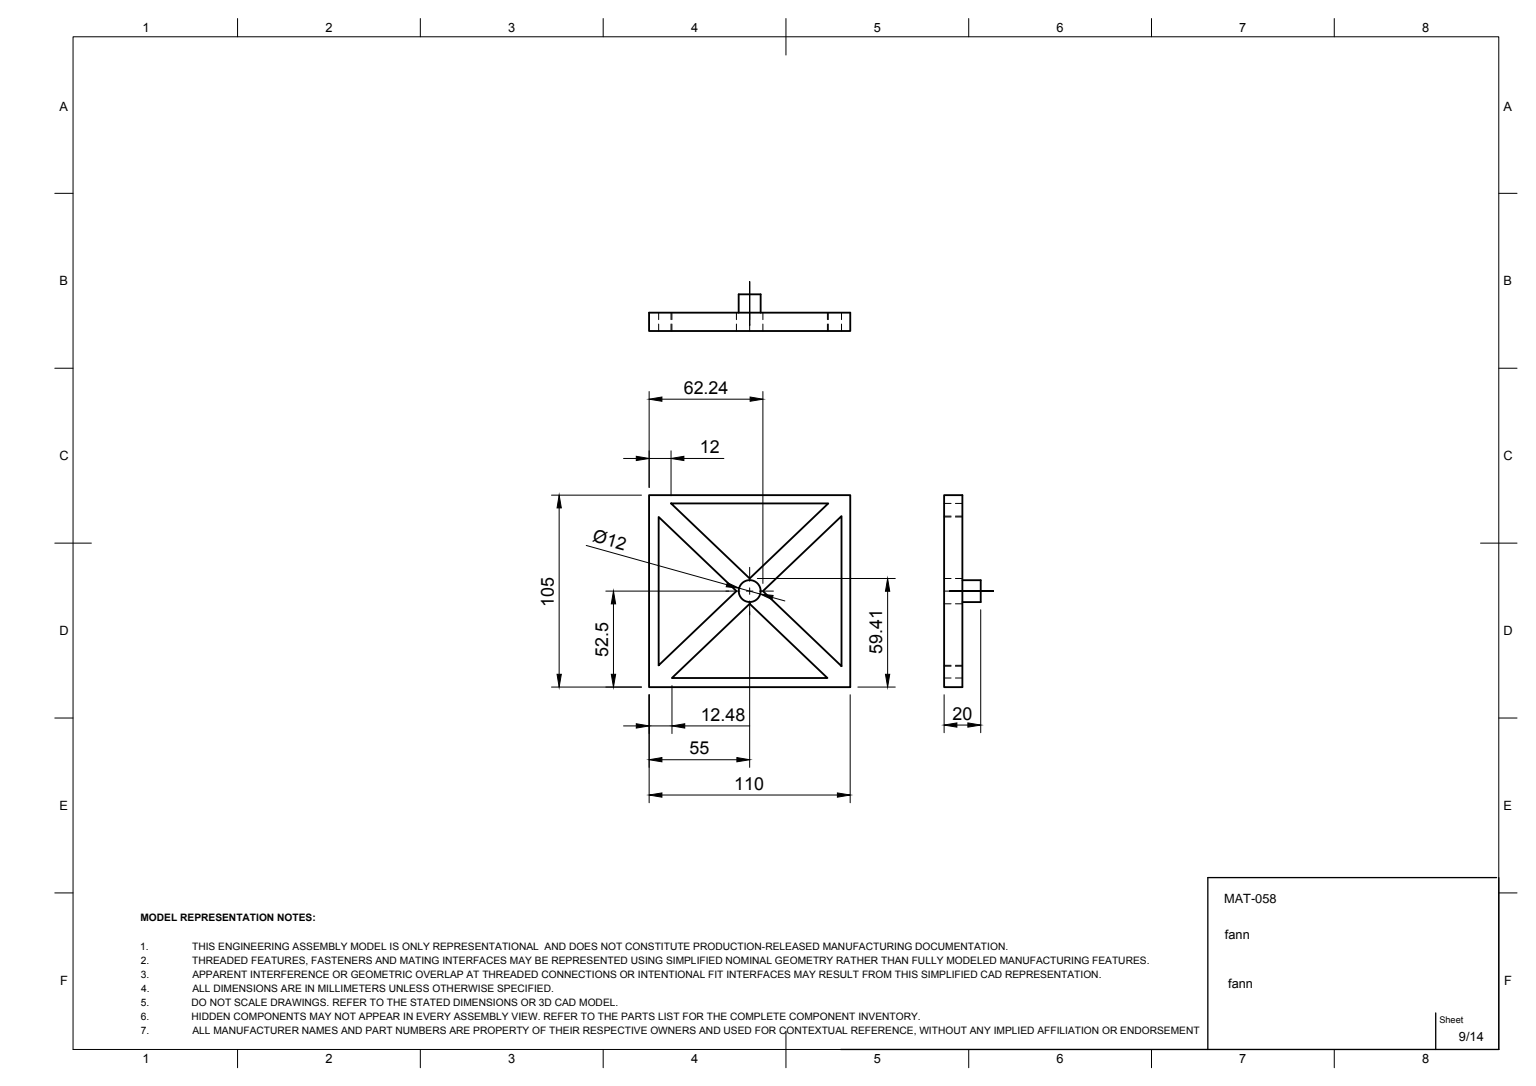
ISO-10303-21;
HEADER;
FILE_DESCRIPTION (('STEP AP214'),
    '1' );
FILE_NAME ('fann.step',
    '2026-10-21T17:54:40',
    ( '' ),
    ( '' ),
    'SwSTEP 2.0',
    'SolidWorks 2026',
    '' );
FILE_SCHEMA (( 'AUTOMOTIVE_DESIGN' ));
ENDSEC;

DATA;
#61=EDGE_LOOP ( 'NONE', ( #36555, #35091, #44528, #47513 ) ) ;
#77=LINE ( 'NONE', #43169, #13986 ) ;
#295=EDGE_CURVE ( 'NONE', #49251, #40145, #37979, .T. ) ;
#419=DIRECTION ( 'NONE',  ( -0.000000000000000000, -0.000000000000000000, -1.000000000000000000 ) ) ;
#426=ORIENTED_EDGE ( 'NONE', *, *, #295, .T. ) ;
#552=AXIS2_PLACEMENT_3D ( 'NONE', #49748, #38283, #46673 ) ;
#596=EDGE_CURVE ( 'NONE', #45670, #46289, #13721, .T. ) ;
#769=CARTESIAN_POINT ( 'NONE',  ( -6.000000000000000888, 0.000000000000000000, 15.00000000000000000 ) ) ;
#797=CARTESIAN_POINT ( 'NONE',  ( 1.040834085586084257E-14, -6.912230148066169200, 5.000000000000000000 ) ) ;
#1005=DIRECTION ( 'NONE',  ( -0.000000000000000000, -0.000000000000000000, -1.000000000000000000 ) ) ;
#1111=LINE ( 'NONE', #9059, #11588 ) ;
#1186=FACE_BOUND ( 'NONE', #10121, .T. ) ;
#1213=EDGE_LOOP ( 'NONE', ( #23628, #22154, #10733 ) ) ;
#1266=EDGE_LOOP ( 'NONE', ( #10992, #14682, #46915, #45929 ) ) ;
#1284=VECTOR ( 'NONE', #35273, 1000.000000000000000 ) ;
#1287=DIRECTION ( 'NONE',  ( 1.000000000000000000, 0.000000000000000000, 0.000000000000000000 ) ) ;
#1333=LINE ( 'NONE', #12605, #28974 ) ;
#1507=EDGE_CURVE ( 'NONE', #2019, #46289, #11808, .T. ) ;
#1571=EDGE_CURVE ( 'NONE', #23819, #8288, #25666, .T. ) ;
#1580=LINE ( 'NONE', #41075, #49952 ) ;
#1585=ORIENTED_EDGE ( 'NONE', *, *, #10780, .F. ) ;
#1661=ORIENTED_EDGE ( 'NONE', *, *, #43378, .T. ) ;
#1783=LINE ( 'NONE', #33099, #13291 ) ;
#1784=ADVANCED_FACE ( 'NONE', ( #43576 ), #5072, .T. ) ;
#1818=CARTESIAN_POINT ( 'NONE',  ( -42.51732812238059722, -47.49695244670218131, 5.000000000000000000 ) ) ;
#2019=VERTEX_POINT ( 'NONE', #22997 ) ;
#2037=CARTESIAN_POINT ( 'NONE',  ( 42.99990394833793061, 47.95759300784327905, -5.000000000000000000 ) ) ;
#2053=CARTESIAN_POINT ( 'NONE',  ( -7.241383964640739634, -3.469446951953614189E-15, -5.000000000000000000 ) ) ;
#2237=CARTESIAN_POINT ( 'NONE',  ( 50.24128791297869867, 41.04536285977714982, 5.000000000000000000 ) ) ;
#2367=( LENGTH_UNIT ( ) NAMED_UNIT ( * ) SI_UNIT ( .MILLI., .METRE. ) );
#2442=LINE ( 'NONE', #49831, #6222 ) ;
#2489=CARTESIAN_POINT ( 'NONE',  ( 55.00000000000002132, -52.50000000000000711, 5.000000000000000000 ) ) ;
#2587=CIRCLE ( 'NONE', #50049, 6.000000000000000888 ) ;
#2625=CARTESIAN_POINT ( 'NONE',  ( 1.040834085586084257E-14, -6.912230148066169200, -5.000000000000000000 ) ) ;
#2888=VECTOR ( 'NONE', #14296, 1000.000000000000000 ) ;
#2900=VERTEX_POINT ( 'NONE', #45837 ) ;
#2966=CARTESIAN_POINT ( 'NONE',  ( -7.241383964640739634, -3.035766082959412415E-15, -5.000000000000000000 ) ) ;
#3027=PLANE ( 'NONE',  #15241 ) ;
#3038=VERTEX_POINT ( 'NONE', #6505 ) ;
#3196=LINE ( 'NONE', #22215, #30009 ) ;
#3263=ORIENTED_EDGE ( 'NONE', *, *, #9906, .T. ) ;
#3280=CARTESIAN_POINT ( 'NONE',  ( 0.000000000000000000, 6.912230148066162094, 5.000000000000000000 ) ) ;
#3429=DIRECTION ( 'NONE',  ( -0.6904757466825005574, 0.7233555441435721711, 0.000000000000000000 ) ) ;
#3501=VECTOR ( 'NONE', #35907, 1000.000000000000000 ) ;
#3639=CARTESIAN_POINT ( 'NONE',  ( 42.51732812238058301, -47.49695244670218131, -5.000000000000000000 ) ) ;
#3650=ORIENTED_EDGE ( 'NONE', *, *, #46157, .T. ) ;
#3868=DIRECTION ( 'NONE',  ( 0.000000000000000000, -0.000000000000000000, 1.000000000000000000 ) ) ;
#3919=EDGE_CURVE ( 'NONE', #7547, #49568, #21277, .T. ) ;
#4033=FACE_OUTER_BOUND ( 'NONE', #36953, .T. ) ;
#4159=ORIENTED_EDGE ( 'NONE', *, *, #3919, .F. ) ;
#4269=PLANE ( 'NONE',  #12903 ) ;
#4290=AXIS2_PLACEMENT_3D ( 'NONE', #33802, #49390, #34296 ) ;
#4292=DIRECTION ( 'NONE',  ( -0.000000000000000000, -0.000000000000000000, -1.000000000000000000 ) ) ;
#4406=AXIS2_PLACEMENT_3D ( 'NONE', #30267, #45123, #10264 ) ;
#4529=AXIS2_PLACEMENT_3D ( 'NONE', #32510, #24796, #12227 ) ;
#4606=DIRECTION ( 'NONE',  ( 0.7233555441435720601, -0.6904757466825006684, 0.000000000000000000 ) ) ;
#4775=ORIENTED_EDGE ( 'NONE', *, *, #30409, .T. ) ;
#4819=DIRECTION ( 'NONE',  ( -0.7233555441435720601, 0.6904757466825006684, 0.000000000000000000 ) ) ;
#4853=CARTESIAN_POINT ( 'NONE',  ( 55.00000000000002132, 52.49999999999999289, -5.000000000000000000 ) ) ;
#5072=PLANE ( 'NONE',  #48594 ) ;
#5077=VECTOR ( 'NONE', #20845, 1000.000000000000000 ) ;
#5159=CIRCLE ( 'NONE', #32211, 6.000000000000000888 ) ;
#5262=ORIENTED_EDGE ( 'NONE', *, *, #43730, .T. ) ;
#5317=ORIENTED_EDGE ( 'NONE', *, *, #18328, .F. ) ;
#5441=ADVANCED_FACE ( 'NONE', ( #26600, #10437, #22490, #10940, #18130, #19136 ), #38165, .F. ) ;
#5621=DIRECTION ( 'NONE',  ( 0.7233555441435720601, 0.6904757466825006684, -0.000000000000000000 ) ) ;
#5698=MANIFOLD_SOLID_BREP ( 'Boss-Extrude2', #36785 ) ;
#6027=LINE ( 'NONE', #48839, #21180 ) ;
#6201=EDGE_CURVE ( 'NONE', #47750, #27906, #24853, .T. ) ;
#6222=VECTOR ( 'NONE', #26300, 1000.000000000000000 ) ;
#6296=ORIENTED_EDGE ( 'NONE', *, *, #12159, .F. ) ;
#6403=DIRECTION ( 'NONE',  ( -0.7233555441435720601, -0.6904757466825006684, 0.000000000000000000 ) ) ;
#6453=ORIENTED_EDGE ( 'NONE', *, *, #12047, .T. ) ;
#6505=CARTESIAN_POINT ( 'NONE',  ( 1.040834085586084257E-14, -6.912230148066169200, 5.000000000000000000 ) ) ;
#6513=ORIENTED_EDGE ( 'NONE', *, *, #36875, .F. ) ;
#6559=VECTOR ( 'NONE', #20961, 1000.000000000000000 ) ;
#6639=APPLICATION_CONTEXT ( 'automotive_design' ) ;
#6641=ORIENTED_EDGE ( 'NONE', *, *, #45637, .T. ) ;
#6674=ORIENTED_EDGE ( 'NONE', *, *, #14486, .F. ) ;
#6715=( NAMED_UNIT ( * ) SI_UNIT ( $, .STERADIAN. ) SOLID_ANGLE_UNIT ( ) );
#7453=DIRECTION ( 'NONE',  ( 0.000000000000000000, 0.000000000000000000, 1.000000000000000000 ) ) ;
#7547=VERTEX_POINT ( 'NONE', #49909 ) ;
#7637=LINE ( 'NONE', #11731, #37690 ) ;
#7709=VECTOR ( 'NONE', #6403, 1000.000000000000000 ) ;
#7722=EDGE_CURVE ( 'NONE', #47029, #47424, #7637, .T. ) ;
#7813=DIRECTION ( 'NONE',  ( 0.000000000000000000, 0.000000000000000000, 1.000000000000000000 ) ) ;
#7815=DIRECTION ( 'NONE',  ( -0.7233555441435721711, -0.6904757466825005574, 0.000000000000000000 ) ) ;
#7881=LINE ( 'NONE', #42739, #9483 ) ;
#7939=APPLICATION_CONTEXT ( 'automotive_design' ) ;
#7988=CARTESIAN_POINT ( 'NONE',  ( -54.99999999999997868, -52.50000000000000711, 5.000000000000000000 ) ) ;
#8037=CARTESIAN_POINT ( 'NONE',  ( 7.241383964640743187, 3.469446951953614189E-15, 5.000000000000000000 ) ) ;
#8204=CIRCLE ( 'NONE', #27053, 6.000000000000000888 ) ;
#8223=CARTESIAN_POINT ( 'NONE',  ( -54.99999999999997868, -52.50000000000000711, -5.000000000000000000 ) ) ;
#8229=VECTOR ( 'NONE', #16574, 1000.000000000000000 ) ;
#8288=VERTEX_POINT ( 'NONE', #37822 ) ;
#8310=PRODUCT_DEFINITION_CONTEXT ( 'detailed design', #6639, 'design' ) ;
#8439=( GEOMETRIC_REPRESENTATION_CONTEXT ( 3 ) GLOBAL_UNCERTAINTY_ASSIGNED_CONTEXT ( ( #36415 ) ) GLOBAL_UNIT_ASSIGNED_CONTEXT ( ( #26535, #13963, #21932 ) ) REPRESENTATION_CONTEXT ( 'NONE', 'WORKASPACE' ) );
#8477=VECTOR ( 'NONE', #25850, 1000.000000000000000 ) ;
#8591=ADVANCED_FACE ( 'NONE', ( #16484 ), #36503, .T. ) ;
#8698=EDGE_CURVE ( 'NONE', #45670, #35747, #8204, .T. ) ;
#8983=ORIENTED_EDGE ( 'NONE', *, *, #1571, .F. ) ;
#9025=EDGE_CURVE ( 'NONE', #42729, #3038, #10721, .T. ) ;
#9038=EDGE_CURVE ( 'NONE', #28813, #31501, #34593, .T. ) ;
#9059=CARTESIAN_POINT ( 'NONE',  ( -42.99990394833793061, 47.95759300784327905, -5.000000000000000000 ) ) ;
#9136=FACE_OUTER_BOUND ( 'NONE', #16855, .T. ) ;
#9184=CARTESIAN_POINT ( 'NONE',  ( -42.99990394833793061, 47.95759300784327905, 5.000000000000000000 ) ) ;
#9188=VERTEX_POINT ( 'NONE', #3639 ) ;
#9235=LINE ( 'NONE', #13588, #25757 ) ;
#9354=FACE_OUTER_BOUND ( 'NONE', #22221, .T. ) ;
#9372=FACE_BOUND ( 'NONE', #47219, .T. ) ;
#9483=VECTOR ( 'NONE', #15054, 1000.000000000000000 ) ;
#9517=LINE ( 'NONE', #25176, #17512 ) ;
#9739=DIRECTION ( 'NONE',  ( -0.7233555441435719491, 0.6904757466825007794, -0.000000000000000000 ) ) ;
#9824=VERTEX_POINT ( 'NONE', #13746 ) ;
#9906=EDGE_CURVE ( 'NONE', #47750, #47029, #3196, .T. ) ;
#9946=EDGE_LOOP ( 'NONE', ( #39923, #4159, #37574, #33449 ) ) ;
#10121=EDGE_LOOP ( 'NONE', ( #426, #3650, #29424 ) ) ;
#10165=ORIENTED_EDGE ( 'NONE', *, *, #1507, .F. ) ;
#10195=CARTESIAN_POINT ( 'NONE',  ( 50.24128791297869867, 41.04536285977714982, 5.000000000000000000 ) ) ;
#10219=ORIENTED_EDGE ( 'NONE', *, *, #45226, .T. ) ;
#10264=DIRECTION ( 'NONE',  ( 1.000000000000000000, 0.000000000000000000, 0.000000000000000000 ) ) ;
#10316=CARTESIAN_POINT ( 'NONE',  ( 0.000000000000000000, 6.912230148066162094, 5.000000000000000000 ) ) ;
#10341=PLANE ( 'NONE',  #31545 ) ;
#10369=VECTOR ( 'NONE', #9739, 1000.000000000000000 ) ;
#10437=FACE_BOUND ( 'NONE', #1213, .T. ) ;
#10445=ADVANCED_FACE ( 'NONE', ( #42651 ), #50567, .T. ) ;
#10468=ADVANCED_FACE ( 'NONE', ( #27277 ), #23158, .F. ) ;
#10573=DIRECTION ( 'NONE',  ( -0.6904757466825006684, 0.7233555441435720601, 0.000000000000000000 ) ) ;
#10720=DIRECTION ( 'NONE',  ( -0.000000000000000000, -0.000000000000000000, -1.000000000000000000 ) ) ;
#10721=LINE ( 'NONE', #20134, #43341 ) ;
#10733=ORIENTED_EDGE ( 'NONE', *, *, #9038, .F. ) ;
#10780=EDGE_CURVE ( 'NONE', #48126, #38712, #15659, .T. ) ;
#10813=EDGE_CURVE ( 'NONE', #47424, #49568, #47174, .T. ) ;
#10828=DIRECTION ( 'NONE',  ( -0.7233555441435720601, -0.6904757466825006684, 0.000000000000000000 ) ) ;
#10940=FACE_OUTER_BOUND ( 'NONE', #31001, .T. ) ;
#10992=ORIENTED_EDGE ( 'NONE', *, *, #43931, .T. ) ;
#11341=CARTESIAN_POINT ( 'NONE',  ( -49.75871208702130133, 40.58472229863599523, -5.000000000000000000 ) ) ;
#11448=ORIENTED_EDGE ( 'NONE', *, *, #29146, .T. ) ;
#11588=VECTOR ( 'NONE', #16752, 1000.000000000000000 ) ;
#11611=CARTESIAN_POINT ( 'NONE',  ( -54.99999999999997868, 52.49999999999999289, 5.000000000000000000 ) ) ;
#11643=DIRECTION ( 'NONE',  ( -0.000000000000000000, -0.000000000000000000, -1.000000000000000000 ) ) ;
#11731=CARTESIAN_POINT ( 'NONE',  ( -54.99999999999997868, 52.49999999999999289, 5.000000000000000000 ) ) ;
#11754=CARTESIAN_POINT ( 'NONE',  ( 50.24128791297869867, 41.04536285977714982, 5.000000000000000000 ) ) ;
#11794=CARTESIAN_POINT ( 'NONE',  ( -42.99990394833793772, 47.95759300784327905, 5.000000000000000000 ) ) ;
#11808=CIRCLE ( 'NONE', #4406, 6.000000000000000888 ) ;
#11837=AXIS2_PLACEMENT_3D ( 'NONE', #45600, #10720, #37693 ) ;
#11880=VECTOR ( 'NONE', #419, 1000.000000000000000 ) ;
#12047=EDGE_CURVE ( 'NONE', #25327, #16502, #36196, .T. ) ;
#12055=ORIENTED_EDGE ( 'NONE', *, *, #43931, .F. ) ;
#12083=PLANE ( 'NONE',  #22647 ) ;
#12091=PLANE ( 'NONE',  #12779 ) ;
#12159=EDGE_CURVE ( 'NONE', #18070, #23819, #17437, .T. ) ;
#12227=DIRECTION ( 'NONE',  ( 0.7233555441435719491, -0.6904757466825007794, 0.000000000000000000 ) ) ;
#12518=LINE ( 'NONE', #47886, #22239 ) ;
#12605=CARTESIAN_POINT ( 'NONE',  ( -7.241383964640739634, -3.469446951953614189E-15, 5.000000000000000000 ) ) ;
#12779=AXIS2_PLACEMENT_3D ( 'NONE', #797, #44122, #35458 ) ;
#12795=CARTESIAN_POINT ( 'NONE',  ( 55.00000000000002132, 52.49999999999999289, 5.000000000000000000 ) ) ;
#12830=CARTESIAN_POINT ( 'NONE',  ( 50.24128791297869867, 41.04536285977714982, -5.000000000000000000 ) ) ;
#12903=AXIS2_PLACEMENT_3D ( 'NONE', #16070, #35846, #24785 ) ;
#13100=PLANE ( 'NONE',  #31081 ) ;
#13291=VECTOR ( 'NONE', #1287, 1000.000000000000000 ) ;
#13378=ORIENTED_EDGE ( 'NONE', *, *, #31800, .T. ) ;
#13523=LINE ( 'NONE', #2237, #22755 ) ;
#13588=CARTESIAN_POINT ( 'NONE',  ( -42.51732812238059722, -47.49695244670218131, -5.000000000000000000 ) ) ;
#13655=CARTESIAN_POINT ( 'NONE',  ( 42.99990394833793061, 47.95759300784327905, 5.000000000000000000 ) ) ;
#13721=LINE ( 'NONE', #48578, #8229 ) ;
#13746=CARTESIAN_POINT ( 'NONE',  ( 0.000000000000000000, 6.912230148066165647, -5.000000000000000000 ) ) ;
#13843=FACE_OUTER_BOUND ( 'NONE', #61, .T. ) ;
#13865=ORIENTED_EDGE ( 'NONE', *, *, #3919, .T. ) ;
#13959=VECTOR ( 'NONE', #1005, 1000.000000000000000 ) ;
#13963=( NAMED_UNIT ( * ) PLANE_ANGLE_UNIT ( ) SI_UNIT ( $, .RADIAN. ) );
#13986=VECTOR ( 'NONE', #19808, 1000.000000000000000 ) ;
#14103=DIRECTION ( 'NONE',  ( 0.000000000000000000, -1.000000000000000000, 0.000000000000000000 ) ) ;
#14189=PLANE ( 'NONE',  #41471 ) ;
#14240=EDGE_CURVE ( 'NONE', #38712, #29224, #24856, .T. ) ;
#14248=ORIENTED_EDGE ( 'NONE', *, *, #35127, .T. ) ;
#14296=DIRECTION ( 'NONE',  ( 0.000000000000000000, 1.000000000000000000, 0.000000000000000000 ) ) ;
#14303=ORIENTED_EDGE ( 'NONE', *, *, #36176, .T. ) ;
#14482=DIRECTION ( 'NONE',  ( 0.000000000000000000, 0.000000000000000000, -1.000000000000000000 ) ) ;
#14486=EDGE_CURVE ( 'NONE', #18872, #49251, #46339, .T. ) ;
#14603=ORIENTED_EDGE ( 'NONE', *, *, #31934, .T. ) ;
#14626=DIRECTION ( 'NONE',  ( -1.000000000000000000, 0.000000000000000000, 0.000000000000000000 ) ) ;
#14682=ORIENTED_EDGE ( 'NONE', *, *, #7722, .F. ) ;
#14896=CARTESIAN_POINT ( 'NONE',  ( 0.000000000000000000, 0.000000000000000000, 15.00000000000000000 ) ) ;
#15054=DIRECTION ( 'NONE',  ( -0.000000000000000000, -0.000000000000000000, -1.000000000000000000 ) ) ;
#15148=DIRECTION ( 'NONE',  ( 0.000000000000000000, 0.000000000000000000, 1.000000000000000000 ) ) ;
#15241=AXIS2_PLACEMENT_3D ( 'NONE', #11754, #49930, #47105 ) ;
#15257=CARTESIAN_POINT ( 'NONE',  ( -42.99990394833793061, 47.95759300784327905, 5.000000000000000000 ) ) ;
#15363=ORIENTED_EDGE ( 'NONE', *, *, #14240, .T. ) ;
#15378=DIRECTION ( 'NONE',  ( 1.000000000000000000, 0.000000000000000000, 0.000000000000000000 ) ) ;
#15442=CARTESIAN_POINT ( 'NONE',  ( 42.99990394833793061, 47.95759300784327905, 5.000000000000000000 ) ) ;
#15495=LINE ( 'NONE', #27306, #1284 ) ;
#15579=ORIENTED_EDGE ( 'NONE', *, *, #43730, .F. ) ;
#15655=DIRECTION ( 'NONE',  ( 1.000000000000000000, 0.000000000000000000, 0.000000000000000000 ) ) ;
#15659=LINE ( 'NONE', #15918, #30048 ) ;
#15828=VECTOR ( 'NONE', #18649, 1000.000000000000000 ) ;
#15865=VECTOR ( 'NONE', #38873, 1000.000000000000000 ) ;
#15918=CARTESIAN_POINT ( 'NONE',  ( -42.99990394833793061, 47.95759300784327905, 5.000000000000000000 ) ) ;
#16070=CARTESIAN_POINT ( 'NONE',  ( 0.000000000000000000, 0.000000000000000000, -5.000000000000000000 ) ) ;
#16195=CARTESIAN_POINT ( 'NONE',  ( 7.241383964640743187, 3.469446951953614189E-15, -5.000000000000000000 ) ) ;
#16232=EDGE_CURVE ( 'NONE', #42729, #9188, #38856, .T. ) ;
#16344=EDGE_LOOP ( 'NONE', ( #45709, #39718, #20107, #26584 ) ) ;
#16391=AXIS2_PLACEMENT_3D ( 'NONE', #16982, #43657, #39848 ) ;
#16397=EDGE_CURVE ( 'NONE', #18511, #9824, #1111, .T. ) ;
#16441=EDGE_LOOP ( 'NONE', ( #50230, #15579, #23509, #23143 ) ) ;
#16484=FACE_OUTER_BOUND ( 'NONE', #16344, .T. ) ;
#16494=EDGE_CURVE ( 'NONE', #48126, #33089, #34619, .T. ) ;
#16502=VERTEX_POINT ( 'NONE', #49707 ) ;
#16574=DIRECTION ( 'NONE',  ( -0.000000000000000000, -0.000000000000000000, -1.000000000000000000 ) ) ;
#16598=ORIENTED_EDGE ( 'NONE', *, *, #17379, .F. ) ;
#16629=EDGE_CURVE ( 'NONE', #33089, #18511, #12518, .T. ) ;
#16752=DIRECTION ( 'NONE',  ( 0.7233555441435720601, -0.6904757466825006684, 0.000000000000000000 ) ) ;
#16814=VERTEX_POINT ( 'NONE', #2489 ) ;
#16855=EDGE_LOOP ( 'NONE', ( #35960, #42593, #36468, #19861 ) ) ;
#16982=CARTESIAN_POINT ( 'NONE',  ( -49.75871208702130133, 40.58472229863599523, 5.000000000000000000 ) ) ;
#17000=ORIENTED_EDGE ( 'NONE', *, *, #596, .F. ) ;
#17071=FACE_BOUND ( 'NONE', #25720, .T. ) ;
#17076=ADVANCED_FACE ( 'NONE', ( #25039 ), #28877, .F. ) ;
#17188=EDGE_LOOP ( 'NONE', ( #17568, #29235, #15363, #5262 ) ) ;
#17200=VECTOR ( 'NONE', #38227, 1000.000000000000000 ) ;
#17216=DIRECTION ( 'NONE',  ( 0.000000000000000000, -0.000000000000000000, -1.000000000000000000 ) ) ;
#17240=ORIENTED_EDGE ( 'NONE', *, *, #47108, .F. ) ;
#17274=ADVANCED_FACE ( 'NONE', ( #33996 ), #22685, .F. ) ;
#17347=EDGE_LOOP ( 'NONE', ( #1661, #44789 ) ) ;
#17379=EDGE_CURVE ( 'NONE', #35747, #2019, #15495, .T. ) ;
#17412=ORIENTED_EDGE ( 'NONE', *, *, #45287, .F. ) ;
#17415=EDGE_CURVE ( 'NONE', #38712, #18511, #39619, .T. ) ;
#17437=LINE ( 'NONE', #37709, #17200 ) ;
#17512=VECTOR ( 'NONE', #48968, 1000.000000000000000 ) ;
#17559=EDGE_LOOP ( 'NONE', ( #17000, #33083, #23343, #29731 ) ) ;
#17568=ORIENTED_EDGE ( 'NONE', *, *, #16397, .F. ) ;
#17717=CARTESIAN_POINT ( 'NONE',  ( -42.99990394833793061, 47.95759300784327905, 5.000000000000000000 ) ) ;
#17768=ORIENTED_EDGE ( 'NONE', *, *, #16629, .T. ) ;
#17865=ORIENTED_EDGE ( 'NONE', *, *, #21387, .T. ) ;
#18002=CARTESIAN_POINT ( 'NONE',  ( -49.75871208702130133, 40.58472229863599523, 5.000000000000000000 ) ) ;
#18070=VERTEX_POINT ( 'NONE', #43318 ) ;
#18130=FACE_BOUND ( 'NONE', #46494, .T. ) ;
#18143=CARTESIAN_POINT ( 'NONE',  ( 50.24128791297869867, -41.04536285977715693, 5.000000000000000000 ) ) ;
#18328=EDGE_CURVE ( 'NONE', #31501, #18070, #2442, .T. ) ;
#18385=LINE ( 'NONE', #10195, #8477 ) ;
#18442=DIRECTION ( 'NONE',  ( -0.000000000000000000, -0.000000000000000000, -1.000000000000000000 ) ) ;
#18511=VERTEX_POINT ( 'NONE', #27821 ) ;
#18578=DIRECTION ( 'NONE',  ( -0.000000000000000000, -0.000000000000000000, -1.000000000000000000 ) ) ;
#18649=DIRECTION ( 'NONE',  ( 1.000000000000000000, 0.000000000000000000, 0.000000000000000000 ) ) ;
#18662=ADVANCED_FACE ( 'NONE', ( #33693 ), #10341, .T. ) ;
#18708=VECTOR ( 'NONE', #19599, 1000.000000000000114 ) ;
#18776=LINE ( 'NONE', #2625, #24953 ) ;
#18800=EDGE_LOOP ( 'NONE', ( #44279, #31453, #49755 ) ) ;
#18844=DIRECTION ( 'NONE',  ( -1.000000000000000000, -0.000000000000000000, -0.000000000000000000 ) ) ;
#18872=VERTEX_POINT ( 'NONE', #11341 ) ;
#18884=EDGE_CURVE ( 'NONE', #29224, #48126, #39824, .T. ) ;
#18922=VECTOR ( 'NONE', #18442, 1000.000000000000000 ) ;
#19136=FACE_BOUND ( 'NONE', #18800, .T. ) ;
#19175=VECTOR ( 'NONE', #43906, 1000.000000000000000 ) ;
#19224=CARTESIAN_POINT ( 'NONE',  ( -54.99999999999997868, 52.49999999999999289, -5.000000000000000000 ) ) ;
#19345=PLANE ( 'NONE',  #28483 ) ;
#19543=EDGE_CURVE ( 'NONE', #31501, #2900, #37672, .T. ) ;
#19590=ORIENTED_EDGE ( 'NONE', *, *, #14240, .F. ) ;
#19599=DIRECTION ( 'NONE',  ( -0.7233555441435721711, -0.6904757466825004464, 0.000000000000000000 ) ) ;
#19665=CARTESIAN_POINT ( 'NONE',  ( 6.000000000000000888, 7.347880794884120722E-16, 15.00000000000000000 ) ) ;
#19677=ADVANCED_FACE ( 'NONE', ( #9136 ), #39695, .T. ) ;
#19683=CYLINDRICAL_SURFACE ( 'NONE', #50185, 6.000000000000000888 ) ;
#19720=DIRECTION ( 'NONE',  ( -1.000000000000000000, -0.000000000000000000, -0.000000000000000000 ) ) ;
#19808=DIRECTION ( 'NONE',  ( -0.000000000000000000, -1.000000000000000000, -0.000000000000000000 ) ) ;
#19819=CARTESIAN_POINT ( 'NONE',  ( -54.99999999999997868, -52.50000000000000711, -5.000000000000000000 ) ) ;
#19861=ORIENTED_EDGE ( 'NONE', *, *, #47108, .T. ) ;
#19929=DIRECTION ( 'NONE',  ( -1.000000000000000000, 0.000000000000000000, 0.000000000000000000 ) ) ;
#19996=AXIS2_PLACEMENT_3D ( 'NONE', #45647, #14626, #7453 ) ;
#20107=ORIENTED_EDGE ( 'NONE', *, *, #37768, .T. ) ;
#20134=CARTESIAN_POINT ( 'NONE',  ( 1.040834085586084257E-14, -6.912230148066169200, 5.000000000000000000 ) ) ;
#20140=ORIENTED_EDGE ( 'NONE', *, *, #42232, .T. ) ;
#20185=ORIENTED_EDGE ( 'NONE', *, *, #18328, .T. ) ;
#20239=LINE ( 'NONE', #39502, #3501 ) ;
#20291=ORIENTED_EDGE ( 'NONE', *, *, #21387, .F. ) ;
#20735=DIRECTION ( 'NONE',  ( 0.6904757466825006684, 0.7233555441435720601, -0.000000000000000000 ) ) ;
#20767=ORIENTED_EDGE ( 'NONE', *, *, #45029, .F. ) ;
#20829=ADVANCED_FACE ( 'NONE', ( #28241 ), #12083, .F. ) ;
#20845=DIRECTION ( 'NONE',  ( -0.000000000000000000, -0.000000000000000000, -1.000000000000000000 ) ) ;
#20961=DIRECTION ( 'NONE',  ( 0.000000000000000000, 1.000000000000000000, 0.000000000000000000 ) ) ;
#21027=AXIS2_PLACEMENT_3D ( 'NONE', #38837, #42905, #39095 ) ;
#21046=LINE ( 'NONE', #36730, #10369 ) ;
#21180=VECTOR ( 'NONE', #18578, 1000.000000000000000 ) ;
#21277=LINE ( 'NONE', #29737, #22058 ) ;
#21346=LINE ( 'NONE', #10316, #5077 ) ;
#21387=EDGE_CURVE ( 'NONE', #32533, #43849, #38604, .T. ) ;
#21475=DIRECTION ( 'NONE',  ( -0.7233555441435720601, -0.6904757466825006684, 0.000000000000000000 ) ) ;
#21735=ADVANCED_FACE ( 'NONE', ( #47948 ), #12091, .T. ) ;
#21889=EDGE_CURVE ( 'NONE', #9188, #29536, #21046, .T. ) ;
#21932=( NAMED_UNIT ( * ) SI_UNIT ( $, .STERADIAN. ) SOLID_ANGLE_UNIT ( ) );
#21946=DIRECTION ( 'NONE',  ( 1.000000000000000000, 0.000000000000000000, -0.000000000000000000 ) ) ;
#22058=VECTOR ( 'NONE', #25386, 1000.000000000000000 ) ;
#22154=ORIENTED_EDGE ( 'NONE', *, *, #19543, .F. ) ;
#22215=CARTESIAN_POINT ( 'NONE',  ( -54.99999999999997868, 52.49999999999999289, 5.000000000000000000 ) ) ;
#22217=ORIENTED_EDGE ( 'NONE', *, *, #45287, .T. ) ;
#22221=EDGE_LOOP ( 'NONE', ( #6674, #31322, #6453, #20140 ) ) ;
#22239=VECTOR ( 'NONE', #19720, 1000.000000000000000 ) ;
#22305=CARTESIAN_POINT ( 'NONE',  ( 50.24128791297869867, 41.04536285977714982, -5.000000000000000000 ) ) ;
#22308=CARTESIAN_POINT ( 'NONE',  ( 6.000000000000000888, 7.347880794884120722E-16, 5.000000000000000000 ) ) ;
#22311=DIRECTION ( 'NONE',  ( 1.000000000000000000, 0.000000000000000000, 0.000000000000000000 ) ) ;
#22430=CARTESIAN_POINT ( 'NONE',  ( -7.241383964640739634, -3.469446951953614189E-15, 5.000000000000000000 ) ) ;
#22490=FACE_BOUND ( 'NONE', #31319, .T. ) ;
#22525=CYLINDRICAL_SURFACE ( 'NONE', #11837, 6.000000000000000888 ) ;
#22647=AXIS2_PLACEMENT_3D ( 'NONE', #7988, #35451, #3868 ) ;
#22683=ADVANCED_FACE ( 'NONE', ( #38217 ), #3027, .T. ) ;
#22685=PLANE ( 'NONE',  #26113 ) ;
#22692=CARTESIAN_POINT ( 'NONE',  ( 1.040834085586084257E-14, -6.912230148066169200, 5.000000000000000000 ) ) ;
#22755=VECTOR ( 'NONE', #21475, 1000.000000000000000 ) ;
#22818=CARTESIAN_POINT ( 'NONE',  ( 0.000000000000000000, 0.000000000000000000, 15.00000000000000000 ) ) ;
#22831=FACE_OUTER_BOUND ( 'NONE', #32878, .T. ) ;
#22925=DIRECTION ( 'NONE',  ( -0.000000000000000000, -0.000000000000000000, -1.000000000000000000 ) ) ;
#22997=CARTESIAN_POINT ( 'NONE',  ( -6.000000000000000888, 0.000000000000000000, 5.000000000000000000 ) ) ;
#23046=EDGE_LOOP ( 'NONE', ( #42458, #11448, #17768 ) ) ;
#23102=PLANE ( 'NONE',  #552 ) ;
#23143=ORIENTED_EDGE ( 'NONE', *, *, #16494, .T. ) ;
#23158=PLANE ( 'NONE',  #21027 ) ;
#23199=LINE ( 'NONE', #22692, #18708 ) ;
#23343=ORIENTED_EDGE ( 'NONE', *, *, #17379, .T. ) ;
#23509=ORIENTED_EDGE ( 'NONE', *, *, #18884, .T. ) ;
#23628=ORIENTED_EDGE ( 'NONE', *, *, #30409, .F. ) ;
#23819=VERTEX_POINT ( 'NONE', #12830 ) ;
#23865=ORIENTED_EDGE ( 'NONE', *, *, #39328, .T. ) ;
#24024=FACE_OUTER_BOUND ( 'NONE', #40152, .T. ) ;
#24175=VECTOR ( 'NONE', #46954, 1000.000000000000000 ) ;
#24337=ORIENTED_EDGE ( 'NONE', *, *, #6201, .F. ) ;
#24497=ORIENTED_EDGE ( 'NONE', *, *, #45029, .T. ) ;
#24641=CARTESIAN_POINT ( 'NONE',  ( -49.75871208702130133, -40.58472229863598102, 5.000000000000000000 ) ) ;
#24785=DIRECTION ( 'NONE',  ( -1.000000000000000000, 0.000000000000000000, -0.000000000000000000 ) ) ;
#24796=DIRECTION ( 'NONE',  ( -0.6904757466825007794, -0.7233555441435719491, 0.000000000000000000 ) ) ;
#24853=LINE ( 'NONE', #12795, #13959 ) ;
#24856=LINE ( 'NONE', #32060, #36892 ) ;
#24891=PRODUCT_DEFINITION_SHAPE ( 'NONE', 'NONE',  #44709 ) ;
#24953=VECTOR ( 'NONE', #34459, 1000.000000000000114 ) ;
#24971=ORIENTED_EDGE ( 'NONE', *, *, #18884, .F. ) ;
#25039=FACE_OUTER_BOUND ( 'NONE', #1266, .T. ) ;
#25176=CARTESIAN_POINT ( 'NONE',  ( 55.00000000000002132, -52.50000000000000711, 5.000000000000000000 ) ) ;
#25327=VERTEX_POINT ( 'NONE', #25592 ) ;
#25386=DIRECTION ( 'NONE',  ( -0.000000000000000000, -0.000000000000000000, -1.000000000000000000 ) ) ;
#25503=DIRECTION ( 'NONE',  ( 0.000000000000000000, 0.000000000000000000, -1.000000000000000000 ) ) ;
#25528=DIRECTION ( 'NONE',  ( 0.000000000000000000, -0.000000000000000000, -1.000000000000000000 ) ) ;
#25592=CARTESIAN_POINT ( 'NONE',  ( -49.75871208702130133, 40.58472229863599523, 5.000000000000000000 ) ) ;
#25666=LINE ( 'NONE', #22305, #7709 ) ;
#25720=EDGE_LOOP ( 'NONE', ( #32202, #38795, #37707 ) ) ;
#25724=( NAMED_UNIT ( * ) PLANE_ANGLE_UNIT ( ) SI_UNIT ( $, .RADIAN. ) );
#25757=VECTOR ( 'NONE', #40293, 1000.000000000000000 ) ;
#25850=DIRECTION ( 'NONE',  ( -0.000000000000000000, -0.000000000000000000, -1.000000000000000000 ) ) ;
#26053=PLANE ( 'NONE',  #37718 ) ;
#26113=AXIS2_PLACEMENT_3D ( 'NONE', #26540, #33748, #14482 ) ;
#26180=ORIENTED_EDGE ( 'NONE', *, *, #36176, .F. ) ;
#26300=DIRECTION ( 'NONE',  ( -0.000000000000000000, -0.000000000000000000, -1.000000000000000000 ) ) ;
#26358=CARTESIAN_POINT ( 'NONE',  ( 50.24128791297869867, -41.04536285977715693, 5.000000000000000000 ) ) ;
#26423=ORIENTED_EDGE ( 'NONE', *, *, #40602, .F. ) ;
#26535=( LENGTH_UNIT ( ) NAMED_UNIT ( * ) SI_UNIT ( .MILLI., .METRE. ) );
#26540=CARTESIAN_POINT ( 'NONE',  ( -54.99999999999997868, -52.50000000000000711, 5.000000000000000000 ) ) ;
#26584=ORIENTED_EDGE ( 'NONE', *, *, #41650, .T. ) ;
#26600=FACE_BOUND ( 'NONE', #47006, .T. ) ;
#26914=ORIENTED_EDGE ( 'NONE', *, *, #16232, .T. ) ;
#27011=ORIENTED_EDGE ( 'NONE', *, *, #38922, .T. ) ;
#27050=LINE ( 'NONE', #40309, #15865 ) ;
#27053=AXIS2_PLACEMENT_3D ( 'NONE', #14896, #15148, #15655 ) ;
#27133=CARTESIAN_POINT ( 'NONE',  ( -49.75871208702130133, -40.58472229863598102, -5.000000000000000000 ) ) ;
#27277=FACE_OUTER_BOUND ( 'NONE', #41458, .T. ) ;
#27306=CARTESIAN_POINT ( 'NONE',  ( -6.000000000000000888, 0.000000000000000000, 15.00000000000000000 ) ) ;
#27385=DIRECTION ( 'NONE',  ( -0.000000000000000000, -1.000000000000000000, -0.000000000000000000 ) ) ;
#27387=DIRECTION ( 'NONE',  ( -0.000000000000000000, -0.000000000000000000, -1.000000000000000000 ) ) ;
#27517=LINE ( 'NONE', #47471, #19175 ) ;
#27778=DIRECTION ( 'NONE',  ( 0.6904757466825007794, 0.7233555441435720601, -0.000000000000000000 ) ) ;
#27821=CARTESIAN_POINT ( 'NONE',  ( -42.99990394833793061, 47.95759300784327905, -5.000000000000000000 ) ) ;
#27906=VERTEX_POINT ( 'NONE', #4853 ) ;
#27918=ORIENTED_EDGE ( 'NONE', *, *, #39438, .F. ) ;
#28241=FACE_OUTER_BOUND ( 'NONE', #39730, .T. ) ;
#28273=DIRECTION ( 'NONE',  ( 0.7233555441435721711, 0.6904757466825005574, -0.000000000000000000 ) ) ;
#28323=VECTOR ( 'NONE', #30778, 1000.000000000000000 ) ;
#28343=ADVANCED_FACE ( 'NONE', ( #9354 ), #14189, .T. ) ;
#28483=AXIS2_PLACEMENT_3D ( 'NONE', #22430, #3429, #7815 ) ;
#28504=PRODUCT_CONTEXT ( 'NONE', #7939, 'mechanical' ) ;
#28613=FACE_BOUND ( 'NONE', #23046, .T. ) ;
#28654=LINE ( 'NONE', #28909, #6559 ) ;
#28775=ORIENTED_EDGE ( 'NONE', *, *, #45637, .F. ) ;
#28776=ADVANCED_FACE ( 'NONE', ( #38018 ), #23102, .T. ) ;
#28813=VERTEX_POINT ( 'NONE', #49501 ) ;
#28852=DIRECTION ( 'NONE',  ( 1.000000000000000000, 0.000000000000000000, 0.000000000000000000 ) ) ;
#28877=PLANE ( 'NONE',  #29416 ) ;
#28909=CARTESIAN_POINT ( 'NONE',  ( 55.00000000000002132, -52.50000000000000711, -5.000000000000000000 ) ) ;
#28974=VECTOR ( 'NONE', #28273, 1000.000000000000114 ) ;
#28978=LINE ( 'NONE', #2037, #45582 ) ;
#29146=EDGE_CURVE ( 'NONE', #9824, #33089, #28978, .T. ) ;
#29224=VERTEX_POINT ( 'NONE', #3280 ) ;
#29235=ORIENTED_EDGE ( 'NONE', *, *, #17415, .F. ) ;
#29282=EDGE_LOOP ( 'NONE', ( #49819, #17240, #14603, #17865 ) ) ;
#29416=AXIS2_PLACEMENT_3D ( 'NONE', #44499, #44755, #25528 ) ;
#29424=ORIENTED_EDGE ( 'NONE', *, *, #14486, .T. ) ;
#29536=VERTEX_POINT ( 'NONE', #32782 ) ;
#29731=ORIENTED_EDGE ( 'NONE', *, *, #1507, .T. ) ;
#29737=CARTESIAN_POINT ( 'NONE',  ( -54.99999999999997868, -52.50000000000000711, 5.000000000000000000 ) ) ;
#29876=EDGE_LOOP ( 'NONE', ( #8983, #28775, #4775, #37336 ) ) ;
#29878=ORIENTED_EDGE ( 'NONE', *, *, #596, .T. ) ;
#29968=ORIENTED_EDGE ( 'NONE', *, *, #31934, .F. ) ;
#29969=LINE ( 'NONE', #38435, #15828 ) ;
#30009=VECTOR ( 'NONE', #18844, 1000.000000000000000 ) ;
#30048=VECTOR ( 'NONE', #43111, 1000.000000000000000 ) ;
#30075=DIRECTION ( 'NONE',  ( -1.000000000000000000, -0.000000000000000000, -0.000000000000000000 ) ) ;
#30263=CARTESIAN_POINT ( 'NONE',  ( -54.99999999999997868, -52.50000000000000711, -5.000000000000000000 ) ) ;
#30267=CARTESIAN_POINT ( 'NONE',  ( 0.000000000000000000, 0.000000000000000000, 5.000000000000000000 ) ) ;
#30409=EDGE_CURVE ( 'NONE', #2900, #28813, #13523, .T. ) ;
#30635=ADVANCED_FACE ( 'NONE', ( #24024, #28613, #17071, #9372, #1186 ), #4269, .T. ) ;
#30710=CARTESIAN_POINT ( 'NONE',  ( 7.241383964640743187, 3.469446951953614189E-15, 5.000000000000000000 ) ) ;
#30778=DIRECTION ( 'NONE',  ( -0.000000000000000000, -0.000000000000000000, -1.000000000000000000 ) ) ;
#30872=ADVANCED_FACE ( 'NONE', ( #41937 ), #19345, .T. ) ;
#30932=CARTESIAN_POINT ( 'NONE',  ( 0.000000000000000000, 0.000000000000000000, 15.00000000000000000 ) ) ;
#31001=EDGE_LOOP ( 'NONE', ( #37450, #3263, #14248, #31772 ) ) ;
#31081=AXIS2_PLACEMENT_3D ( 'NONE', #17717, #14103, #17216 ) ;
#31111=VECTOR ( 'NONE', #27385, 1000.000000000000000 ) ;
#31319=EDGE_LOOP ( 'NONE', ( #24971, #19590, #1585 ) ) ;
#31322=ORIENTED_EDGE ( 'NONE', *, *, #41650, .F. ) ;
#31453=ORIENTED_EDGE ( 'NONE', *, *, #39328, .F. ) ;
#31501=VERTEX_POINT ( 'NONE', #26358 ) ;
#31545=AXIS2_PLACEMENT_3D ( 'NONE', #45695, #10573, #10828 ) ;
#31712=DIRECTION ( 'NONE',  ( -0.7233555441435719491, 0.6904757466825007794, -0.000000000000000000 ) ) ;
#31772=ORIENTED_EDGE ( 'NONE', *, *, #36875, .T. ) ;
#31800=EDGE_CURVE ( 'NONE', #40868, #40145, #6027, .T. ) ;
#31923=CARTESIAN_POINT ( 'NONE',  ( 0.000000000000000000, 0.000000000000000000, 0.000000000000000000 ) ) ;
#31933=CARTESIAN_POINT ( 'NONE',  ( 42.51732812238058301, -47.49695244670218131, 5.000000000000000000 ) ) ;
#31934=EDGE_CURVE ( 'NONE', #3038, #32533, #23199, .T. ) ;
#31958=CARTESIAN_POINT ( 'NONE',  ( -49.75871208702130133, -40.58472229863598102, -5.000000000000000000 ) ) ;
#32060=CARTESIAN_POINT ( 'NONE',  ( -42.99990394833793061, 47.95759300784327905, 5.000000000000000000 ) ) ;
#32097=LINE ( 'NONE', #16195, #37128 ) ;
#32202=ORIENTED_EDGE ( 'NONE', *, *, #46931, .T. ) ;
#32211=AXIS2_PLACEMENT_3D ( 'NONE', #41803, #38731, #15378 ) ;
#32510=CARTESIAN_POINT ( 'NONE',  ( 1.040834085586084257E-14, -6.912230148066169200, 5.000000000000000000 ) ) ;
#32533=VERTEX_POINT ( 'NONE', #1818 ) ;
#32569=ADVANCED_FACE ( 'NONE', ( #13843 ), #13100, .T. ) ;
#32782=CARTESIAN_POINT ( 'NONE',  ( 1.040834085586084257E-14, -6.912230148066169200, -5.000000000000000000 ) ) ;
#32878=EDGE_LOOP ( 'NONE', ( #6296, #5317, #37890, #6641 ) ) ;
#32926=ORIENTED_EDGE ( 'NONE', *, *, #9025, .F. ) ;
#33013=STYLED_ITEM('',(#50782),#5698);
#33083=ORIENTED_EDGE ( 'NONE', *, *, #43378, .F. ) ;
#33089=VERTEX_POINT ( 'NONE', #43215 ) ;
#33099=CARTESIAN_POINT ( 'NONE',  ( -54.99999999999997868, -52.50000000000000711, 5.000000000000000000 ) ) ;
#33111=PRODUCT ( 'fann', 'fann', '', ( #28504 ) ) ;
#33302=ORIENTED_EDGE ( 'NONE', *, *, #38922, .F. ) ;
#33449=ORIENTED_EDGE ( 'NONE', *, *, #7722, .T. ) ;
#33471=CARTESIAN_POINT ( 'NONE',  ( -49.75871208702130133, -40.58472229863598102, 5.000000000000000000 ) ) ;
#33556=ADVANCED_FACE ( 'NONE', ( #41443 ), #26053, .T. ) ;
#33693=FACE_OUTER_BOUND ( 'NONE', #16441, .T. ) ;
#33748=DIRECTION ( 'NONE',  ( 1.000000000000000000, 0.000000000000000000, 0.000000000000000000 ) ) ;
#33802=CARTESIAN_POINT ( 'NONE',  ( 0.000000000000000000, 0.000000000000000000, 5.000000000000000000 ) ) ;
#33920=LINE ( 'NONE', #50010, #37862 ) ;
#33996=FACE_OUTER_BOUND ( 'NONE', #9946, .T. ) ;
#34013=ORIENTED_EDGE ( 'NONE', *, *, #34312, .F. ) ;
#34296=DIRECTION ( 'NONE',  ( -1.000000000000000000, 0.000000000000000000, -0.000000000000000000 ) ) ;
#34312=EDGE_CURVE ( 'NONE', #16814, #34456, #1580, .T. ) ;
#34456=VERTEX_POINT ( 'NONE', #45395 ) ;
#34459=DIRECTION ( 'NONE',  ( -0.7233555441435721711, -0.6904757466825004464, 0.000000000000000000 ) ) ;
#34593=LINE ( 'NONE', #46357, #42531 ) ;
#34619=LINE ( 'NONE', #13655, #18922 ) ;
#34651=PLANE ( 'NONE',  #19996 ) ;
#34661=SHAPE_REPRESENTATION ( 'fann', ( #45486 ), #46291 ) ;
#34662=MECHANICAL_DESIGN_GEOMETRIC_PRESENTATION_REPRESENTATION('',(#33013),#8439);
#35026=DIRECTION ( 'NONE',  ( 1.000000000000000000, 0.000000000000000000, 0.000000000000000000 ) ) ;
#35091=ORIENTED_EDGE ( 'NONE', *, *, #16494, .F. ) ;
#35127=EDGE_CURVE ( 'NONE', #47029, #7547, #77, .T. ) ;
#35183=DIRECTION ( 'NONE',  ( -0.000000000000000000, -1.000000000000000000, -0.000000000000000000 ) ) ;
#35273=DIRECTION ( 'NONE',  ( -0.000000000000000000, -0.000000000000000000, -1.000000000000000000 ) ) ;
#35451=DIRECTION ( 'NONE',  ( 0.000000000000000000, 1.000000000000000000, 0.000000000000000000 ) ) ;
#35458=DIRECTION ( 'NONE',  ( 0.7233555441435721711, 0.6904757466825004464, 0.000000000000000000 ) ) ;
#35733=VECTOR ( 'NONE', #47010, 1000.000000000000000 ) ;
#35741=VECTOR ( 'NONE', #11643, 1000.000000000000000 ) ;
#35747=VERTEX_POINT ( 'NONE', #769 ) ;
#35759=DIRECTION ( 'NONE',  ( -0.7233555441435720601, 0.6904757466825007794, 0.000000000000000000 ) ) ;
#35846=DIRECTION ( 'NONE',  ( 0.000000000000000000, 0.000000000000000000, -1.000000000000000000 ) ) ;
#35863=CARTESIAN_POINT ( 'NONE',  ( 55.00000000000002132, 52.49999999999999289, 5.000000000000000000 ) ) ;
#35907=DIRECTION ( 'NONE',  ( -0.7233555441435720601, 0.6904757466825006684, -0.000000000000000000 ) ) ;
#35948=DIRECTION ( 'NONE',  ( -0.000000000000000000, -1.000000000000000000, -0.000000000000000000 ) ) ;
#35960=ORIENTED_EDGE ( 'NONE', *, *, #21889, .F. ) ;
#35962=SHAPE_DEFINITION_REPRESENTATION ( #24891, #34661 ) ;
#35982=DIRECTION ( 'NONE',  ( -0.000000000000000000, -0.000000000000000000, -1.000000000000000000 ) ) ;
#36176=EDGE_CURVE ( 'NONE', #34456, #27906, #28654, .T. ) ;
#36196=LINE ( 'NONE', #24641, #49912 ) ;
#36415=UNCERTAINTY_MEASURE_WITH_UNIT (LENGTH_MEASURE( 1.000000000000000082E-05 ), #26535, 'distance_accuracy_value', 'NONE');
#36468=ORIENTED_EDGE ( 'NONE', *, *, #9025, .T. ) ;
#36503=PLANE ( 'NONE',  #16391 ) ;
#36507=PRODUCT_DEFINITION_FORMATION_WITH_SPECIFIED_SOURCE ( 'ANY', '', #33111, .NOT_KNOWN. ) ;
#36555=ORIENTED_EDGE ( 'NONE', *, *, #16629, .F. ) ;
#36626=AXIS2_PLACEMENT_3D ( 'NONE', #8037, #27778, #35759 ) ;
#36730=CARTESIAN_POINT ( 'NONE',  ( 1.040834085586084257E-14, -6.912230148066169200, -5.000000000000000000 ) ) ;
#36785=CLOSED_SHELL ( 'NONE', ( #47836, #5441, #30635, #10468, #17076, #17274, #20829, #18662, #32569, #1784, #28776, #19677, #21735, #22683, #10445, #47285, #8591, #28343, #30872, #48749, #33556 ) ) ;
#36809=ORIENTED_EDGE ( 'NONE', *, *, #41208, .F. ) ;
#36875=EDGE_CURVE ( 'NONE', #7547, #16814, #1783, .T. ) ;
#36892=VECTOR ( 'NONE', #4606, 1000.000000000000000 ) ;
#36953=EDGE_LOOP ( 'NONE', ( #43299, #29878, #10219, #16598 ) ) ;
#37128=VECTOR ( 'NONE', #43882, 999.9999999999998863 ) ;
#37285=EDGE_LOOP ( 'NONE', ( #26423, #20291, #27011, #26914 ) ) ;
#37336=ORIENTED_EDGE ( 'NONE', *, *, #41208, .T. ) ;
#37450=ORIENTED_EDGE ( 'NONE', *, *, #39438, .T. ) ;
#37574=ORIENTED_EDGE ( 'NONE', *, *, #35127, .F. ) ;
#37672=LINE ( 'NONE', #18143, #2888 ) ;
#37690=VECTOR ( 'NONE', #27387, 1000.000000000000000 ) ;
#37693=DIRECTION ( 'NONE',  ( -1.000000000000000000, 0.000000000000000000, 0.000000000000000000 ) ) ;
#37707=ORIENTED_EDGE ( 'NONE', *, *, #21889, .T. ) ;
#37709=CARTESIAN_POINT ( 'NONE',  ( 50.24128791297869867, -41.04536285977715693, -5.000000000000000000 ) ) ;
#37718=AXIS2_PLACEMENT_3D ( 'NONE', #30932, #41697, #21946 ) ;
#37768=EDGE_CURVE ( 'NONE', #40868, #25327, #20239, .T. ) ;
#37822=CARTESIAN_POINT ( 'NONE',  ( 7.241383964640743187, 3.469446951953614189E-15, -5.000000000000000000 ) ) ;
#37862=VECTOR ( 'NONE', #30075, 1000.000000000000000 ) ;
#37890=ORIENTED_EDGE ( 'NONE', *, *, #19543, .T. ) ;
#37979=LINE ( 'NONE', #2053, #49838 ) ;
#38018=FACE_OUTER_BOUND ( 'NONE', #37285, .T. ) ;
#38028=CARTESIAN_POINT ( 'NONE',  ( -42.51732812238060433, -47.49695244670218841, -5.000000000000000000 ) ) ;
#38165=PLANE ( 'NONE',  #4290 ) ;
#38217=FACE_OUTER_BOUND ( 'NONE', #29876, .T. ) ;
#38227=DIRECTION ( 'NONE',  ( 0.000000000000000000, 1.000000000000000000, 0.000000000000000000 ) ) ;
#38231=VECTOR ( 'NONE', #35183, 1000.000000000000000 ) ;
#38283=DIRECTION ( 'NONE',  ( 0.000000000000000000, 1.000000000000000000, 0.000000000000000000 ) ) ;
#38302=SHAPE_REPRESENTATION_RELATIONSHIP ( 'NONE' , 'NONE' ,  #34661, #42356 ) ;
#38435=CARTESIAN_POINT ( 'NONE',  ( -42.51732812238059722, -47.49695244670218131, 5.000000000000000000 ) ) ;
#38498=DIRECTION ( 'NONE',  ( 0.000000000000000000, 0.000000000000000000, 1.000000000000000000 ) ) ;
#38587=ORIENTED_EDGE ( 'NONE', *, *, #9038, .T. ) ;
#38604=LINE ( 'NONE', #45987, #35741 ) ;
#38662=LINE ( 'NONE', #30710, #11880 ) ;
#38712=VERTEX_POINT ( 'NONE', #11794 ) ;
#38731=DIRECTION ( 'NONE',  ( 0.000000000000000000, 0.000000000000000000, 1.000000000000000000 ) ) ;
#38795=ORIENTED_EDGE ( 'NONE', *, *, #40602, .T. ) ;
#38831=UNCERTAINTY_MEASURE_WITH_UNIT (LENGTH_MEASURE( 1.000000000000000082E-05 ), #2367, 'distance_accuracy_value', 'NONE');
#38837=CARTESIAN_POINT ( 'NONE',  ( 55.00000000000002132, -52.50000000000000711, 5.000000000000000000 ) ) ;
#38856=LINE ( 'NONE', #43434, #45933 ) ;
#38873=DIRECTION ( 'NONE',  ( -0.7233555441435720601, 0.6904757466825006684, -0.000000000000000000 ) ) ;
#38922=EDGE_CURVE ( 'NONE', #32533, #42729, #29969, .T. ) ;
#39095=DIRECTION ( 'NONE',  ( 0.000000000000000000, 0.000000000000000000, 1.000000000000000000 ) ) ;
#39328=EDGE_CURVE ( 'NONE', #16502, #40868, #1333, .T. ) ;
#39438=EDGE_CURVE ( 'NONE', #16814, #47750, #9517, .T. ) ;
#39502=CARTESIAN_POINT ( 'NONE',  ( -49.75871208702130133, 40.58472229863599523, 5.000000000000000000 ) ) ;
#39619=LINE ( 'NONE', #15257, #35733 ) ;
#39695=PLANE ( 'NONE',  #4529 ) ;
#39718=ORIENTED_EDGE ( 'NONE', *, *, #31800, .F. ) ;
#39730=EDGE_LOOP ( 'NONE', ( #22217, #34013, #6513, #13865 ) ) ;
#39824=LINE ( 'NONE', #15442, #24175 ) ;
#39848=DIRECTION ( 'NONE',  ( 0.7233555441435720601, -0.6904757466825006684, 0.000000000000000000 ) ) ;
#39923=ORIENTED_EDGE ( 'NONE', *, *, #10813, .T. ) ;
#40092=ORIENTED_EDGE ( 'NONE', *, *, #1571, .T. ) ;
#40145=VERTEX_POINT ( 'NONE', #2966 ) ;
#40152=EDGE_LOOP ( 'NONE', ( #26180, #17412, #47463, #12055 ) ) ;
#40293=DIRECTION ( 'NONE',  ( 1.000000000000000000, 0.000000000000000000, 0.000000000000000000 ) ) ;
#40309=CARTESIAN_POINT ( 'NONE',  ( -49.75871208702130133, 40.58472229863599523, -5.000000000000000000 ) ) ;
#40602=EDGE_CURVE ( 'NONE', #43849, #9188, #9235, .T. ) ;
#40868=VERTEX_POINT ( 'NONE', #47124 ) ;
#41051=DIRECTION ( 'NONE',  ( 0.7233555441435721711, 0.6904757466825005574, -0.000000000000000000 ) ) ;
#41075=CARTESIAN_POINT ( 'NONE',  ( 55.00000000000002132, -52.50000000000000711, 5.000000000000000000 ) ) ;
#41208=EDGE_CURVE ( 'NONE', #28813, #8288, #38662, .T. ) ;
#41443=FACE_OUTER_BOUND ( 'NONE', #17347, .T. ) ;
#41458=EDGE_LOOP ( 'NONE', ( #14303, #24337, #27918, #43017 ) ) ;
#41471=AXIS2_PLACEMENT_3D ( 'NONE', #33471, #28852, #25503 ) ;
#41650=EDGE_CURVE ( 'NONE', #25327, #18872, #43442, .T. ) ;
#41697=DIRECTION ( 'NONE',  ( 0.000000000000000000, 0.000000000000000000, 1.000000000000000000 ) ) ;
#41803=CARTESIAN_POINT ( 'NONE',  ( 0.000000000000000000, 0.000000000000000000, 5.000000000000000000 ) ) ;
#41937=FACE_OUTER_BOUND ( 'NONE', #50056, .T. ) ;
#42007=VECTOR ( 'NONE', #50470, 1000.000000000000000 ) ;
#42232=EDGE_CURVE ( 'NONE', #16502, #49251, #7881, .T. ) ;
#42356=ADVANCED_BREP_SHAPE_REPRESENTATION ( '', ( #5698, #45486 ), #46291 ) ;
#42458=ORIENTED_EDGE ( 'NONE', *, *, #16397, .T. ) ;
#42531=VECTOR ( 'NONE', #49923, 999.9999999999998863 ) ;
#42593=ORIENTED_EDGE ( 'NONE', *, *, #16232, .F. ) ;
#42651=FACE_OUTER_BOUND ( 'NONE', #47185, .T. ) ;
#42729=VERTEX_POINT ( 'NONE', #31933 ) ;
#42739=CARTESIAN_POINT ( 'NONE',  ( -49.75871208702130133, -40.58472229863598102, 5.000000000000000000 ) ) ;
#42905=DIRECTION ( 'NONE',  ( -1.000000000000000000, 0.000000000000000000, 0.000000000000000000 ) ) ;
#43017=ORIENTED_EDGE ( 'NONE', *, *, #34312, .T. ) ;
#43111=DIRECTION ( 'NONE',  ( -1.000000000000000000, -0.000000000000000000, -0.000000000000000000 ) ) ;
#43169=CARTESIAN_POINT ( 'NONE',  ( -54.99999999999997868, -52.50000000000000711, 5.000000000000000000 ) ) ;
#43215=CARTESIAN_POINT ( 'NONE',  ( 42.99990394833793061, 47.95759300784327905, -5.000000000000000000 ) ) ;
#43299=ORIENTED_EDGE ( 'NONE', *, *, #8698, .F. ) ;
#43318=CARTESIAN_POINT ( 'NONE',  ( 50.24128791297869867, -41.04536285977715693, -5.000000000000000000 ) ) ;
#43330=ORIENTED_EDGE ( 'NONE', *, *, #295, .F. ) ;
#43341=VECTOR ( 'NONE', #31712, 1000.000000000000000 ) ;
#43378=EDGE_CURVE ( 'NONE', #35747, #45670, #2587, .T. ) ;
#43434=CARTESIAN_POINT ( 'NONE',  ( 42.51732812238058301, -47.49695244670218131, 5.000000000000000000 ) ) ;
#43442=LINE ( 'NONE', #18002, #28323 ) ;
#43576=FACE_OUTER_BOUND ( 'NONE', #17188, .T. ) ;
#43657=DIRECTION ( 'NONE',  ( -0.6904757466825006684, -0.7233555441435720601, 0.000000000000000000 ) ) ;
#43730=EDGE_CURVE ( 'NONE', #29224, #9824, #21346, .T. ) ;
#43849=VERTEX_POINT ( 'NONE', #38028 ) ;
#43882=DIRECTION ( 'NONE',  ( 0.7233555441435720601, -0.6904757466825007794, 0.000000000000000000 ) ) ;
#43906=DIRECTION ( 'NONE',  ( -0.000000000000000000, -0.000000000000000000, -1.000000000000000000 ) ) ;
#43931=EDGE_CURVE ( 'NONE', #27906, #47424, #33920, .T. ) ;
#44122=DIRECTION ( 'NONE',  ( 0.6904757466825005574, -0.7233555441435722821, 0.000000000000000000 ) ) ;
#44157=CARTESIAN_POINT ( 'NONE',  ( 42.99990394833793061, 47.95759300784327905, 5.000000000000000000 ) ) ;
#44279=ORIENTED_EDGE ( 'NONE', *, *, #37768, .F. ) ;
#44326=ORIENTED_EDGE ( 'NONE', *, *, #45226, .F. ) ;
#44499=CARTESIAN_POINT ( 'NONE',  ( -54.99999999999997868, 52.49999999999999289, 5.000000000000000000 ) ) ;
#44528=ORIENTED_EDGE ( 'NONE', *, *, #10780, .T. ) ;
#44709=PRODUCT_DEFINITION ( 'UNKNOWN', '', #36507, #8310 ) ;
#44755=DIRECTION ( 'NONE',  ( 0.000000000000000000, -1.000000000000000000, 0.000000000000000000 ) ) ;
#44789=ORIENTED_EDGE ( 'NONE', *, *, #8698, .T. ) ;
#45029=EDGE_CURVE ( 'NONE', #8288, #18070, #32097, .T. ) ;
#45123=DIRECTION ( 'NONE',  ( 0.000000000000000000, 0.000000000000000000, 1.000000000000000000 ) ) ;
#45226=EDGE_CURVE ( 'NONE', #46289, #2019, #5159, .T. ) ;
#45287=EDGE_CURVE ( 'NONE', #49568, #34456, #45869, .T. ) ;
#45338=FACE_OUTER_BOUND ( 'NONE', #17559, .T. ) ;
#45395=CARTESIAN_POINT ( 'NONE',  ( 55.00000000000002132, -52.50000000000000711, -5.000000000000000000 ) ) ;
#45486=AXIS2_PLACEMENT_3D ( 'NONE', #31923, #7813, #35026 ) ;
#45582=VECTOR ( 'NONE', #5621, 1000.000000000000000 ) ;
#45600=CARTESIAN_POINT ( 'NONE',  ( 0.000000000000000000, 0.000000000000000000, 15.00000000000000000 ) ) ;
#45637=EDGE_CURVE ( 'NONE', #2900, #23819, #18385, .T. ) ;
#45647=CARTESIAN_POINT ( 'NONE',  ( 50.24128791297869867, -41.04536285977715693, 5.000000000000000000 ) ) ;
#45670=VERTEX_POINT ( 'NONE', #19665 ) ;
#45695=CARTESIAN_POINT ( 'NONE',  ( 42.99990394833793061, 47.95759300784327905, 5.000000000000000000 ) ) ;
#45709=ORIENTED_EDGE ( 'NONE', *, *, #46157, .F. ) ;
#45837=CARTESIAN_POINT ( 'NONE',  ( 50.24128791297869867, 41.04536285977714982, 5.000000000000000000 ) ) ;
#45869=LINE ( 'NONE', #30263, #42007 ) ;
#45929=ORIENTED_EDGE ( 'NONE', *, *, #6201, .T. ) ;
#45933=VECTOR ( 'NONE', #22925, 1000.000000000000000 ) ;
#45987=CARTESIAN_POINT ( 'NONE',  ( -42.51732812238059722, -47.49695244670218131, 5.000000000000000000 ) ) ;
#46157=EDGE_CURVE ( 'NONE', #40145, #18872, #27050, .T. ) ;
#46289=VERTEX_POINT ( 'NONE', #22308 ) ;
#46291=( GEOMETRIC_REPRESENTATION_CONTEXT ( 3 ) GLOBAL_UNCERTAINTY_ASSIGNED_CONTEXT ( ( #38831 ) ) GLOBAL_UNIT_ASSIGNED_CONTEXT ( ( #2367, #25724, #6715 ) ) REPRESENTATION_CONTEXT ( 'NONE', 'WORKASPACE' ) );
#46339=LINE ( 'NONE', #27133, #31111 ) ;
#46357=CARTESIAN_POINT ( 'NONE',  ( 7.241383964640743187, 3.469446951953614189E-15, 5.000000000000000000 ) ) ;
#46494=EDGE_LOOP ( 'NONE', ( #33302, #29968, #32926 ) ) ;
#46673=DIRECTION ( 'NONE',  ( 0.000000000000000000, -0.000000000000000000, 1.000000000000000000 ) ) ;
#46915=ORIENTED_EDGE ( 'NONE', *, *, #9906, .F. ) ;
#46931=EDGE_CURVE ( 'NONE', #29536, #43849, #18776, .T. ) ;
#46954=DIRECTION ( 'NONE',  ( 0.7233555441435720601, 0.6904757466825006684, -0.000000000000000000 ) ) ;
#47006=EDGE_LOOP ( 'NONE', ( #10165, #44326 ) ) ;
#47010=DIRECTION ( 'NONE',  ( -0.000000000000000000, -0.000000000000000000, -1.000000000000000000 ) ) ;
#47029=VERTEX_POINT ( 'NONE', #11611 ) ;
#47089=CARTESIAN_POINT ( 'NONE',  ( 0.000000000000000000, 0.000000000000000000, 15.00000000000000000 ) ) ;
#47105=DIRECTION ( 'NONE',  ( 0.7233555441435720601, 0.6904757466825006684, 0.000000000000000000 ) ) ;
#47108=EDGE_CURVE ( 'NONE', #3038, #29536, #27517, .T. ) ;
#47124=CARTESIAN_POINT ( 'NONE',  ( -7.241383964640739634, -3.469446951953614189E-15, 5.000000000000000000 ) ) ;
#47174=LINE ( 'NONE', #8223, #38231 ) ;
#47185=EDGE_LOOP ( 'NONE', ( #20767, #36809, #38587, #20185 ) ) ;
#47219=EDGE_LOOP ( 'NONE', ( #49224, #40092, #24497 ) ) ;
#47285=ADVANCED_FACE ( 'NONE', ( #22831 ), #34651, .T. ) ;
#47424=VERTEX_POINT ( 'NONE', #19224 ) ;
#47463=ORIENTED_EDGE ( 'NONE', *, *, #10813, .F. ) ;
#47471=CARTESIAN_POINT ( 'NONE',  ( 1.040834085586084257E-14, -6.912230148066169200, 5.000000000000000000 ) ) ;
#47513=ORIENTED_EDGE ( 'NONE', *, *, #17415, .T. ) ;
#47750=VERTEX_POINT ( 'NONE', #35863 ) ;
#47836=ADVANCED_FACE ( 'NONE', ( #4033 ), #19683, .T. ) ;
#47886=CARTESIAN_POINT ( 'NONE',  ( -42.99990394833793061, 47.95759300784327905, -5.000000000000000000 ) ) ;
#47948=FACE_OUTER_BOUND ( 'NONE', #29282, .T. ) ;
#48126=VERTEX_POINT ( 'NONE', #44157 ) ;
#48578=CARTESIAN_POINT ( 'NONE',  ( 6.000000000000000888, 7.347880794884120722E-16, 15.00000000000000000 ) ) ;
#48594=AXIS2_PLACEMENT_3D ( 'NONE', #9184, #20735, #4819 ) ;
#48749=ADVANCED_FACE ( 'NONE', ( #45338 ), #22525, .T. ) ;
#48839=CARTESIAN_POINT ( 'NONE',  ( -7.241383964640739634, -3.469446951953614189E-15, 5.000000000000000000 ) ) ;
#48968=DIRECTION ( 'NONE',  ( 0.000000000000000000, 1.000000000000000000, 0.000000000000000000 ) ) ;
#49224=ORIENTED_EDGE ( 'NONE', *, *, #12159, .T. ) ;
#49251=VERTEX_POINT ( 'NONE', #31958 ) ;
#49390=DIRECTION ( 'NONE',  ( 0.000000000000000000, 0.000000000000000000, -1.000000000000000000 ) ) ;
#49501=CARTESIAN_POINT ( 'NONE',  ( 7.241383964640743187, 3.469446951953614189E-15, 5.000000000000000000 ) ) ;
#49568=VERTEX_POINT ( 'NONE', #19819 ) ;
#49707=CARTESIAN_POINT ( 'NONE',  ( -49.75871208702130133, -40.58472229863598102, 5.000000000000000000 ) ) ;
#49748=CARTESIAN_POINT ( 'NONE',  ( -42.51732812238059722, -47.49695244670218131, 5.000000000000000000 ) ) ;
#49755=ORIENTED_EDGE ( 'NONE', *, *, #12047, .F. ) ;
#49819=ORIENTED_EDGE ( 'NONE', *, *, #46931, .F. ) ;
#49831=CARTESIAN_POINT ( 'NONE',  ( 50.24128791297869867, -41.04536285977715693, 5.000000000000000000 ) ) ;
#49838=VECTOR ( 'NONE', #41051, 1000.000000000000114 ) ;
#49909=CARTESIAN_POINT ( 'NONE',  ( -54.99999999999997868, -52.50000000000000711, 5.000000000000000000 ) ) ;
#49912=VECTOR ( 'NONE', #35948, 1000.000000000000000 ) ;
#49923=DIRECTION ( 'NONE',  ( 0.7233555441435720601, -0.6904757466825007794, 0.000000000000000000 ) ) ;
#49930=DIRECTION ( 'NONE',  ( 0.6904757466825006684, -0.7233555441435720601, 0.000000000000000000 ) ) ;
#49952=VECTOR ( 'NONE', #35982, 1000.000000000000000 ) ;
#50010=CARTESIAN_POINT ( 'NONE',  ( -54.99999999999997868, 52.49999999999999289, -5.000000000000000000 ) ) ;
#50049=AXIS2_PLACEMENT_3D ( 'NONE', #22818, #38498, #22311 ) ;
#50056=EDGE_LOOP ( 'NONE', ( #43330, #50446, #23865, #13378 ) ) ;
#50185=AXIS2_PLACEMENT_3D ( 'NONE', #47089, #4292, #19929 ) ;
#50230=ORIENTED_EDGE ( 'NONE', *, *, #29146, .F. ) ;
#50446=ORIENTED_EDGE ( 'NONE', *, *, #42232, .F. ) ;
#50470=DIRECTION ( 'NONE',  ( 1.000000000000000000, 0.000000000000000000, 0.000000000000000000 ) ) ;
#50567=PLANE ( 'NONE',  #36626 ) ;
#50776=COLOUR_RGB('Off White',0.89,0.88,0.83);
#50777=FILL_AREA_STYLE_COLOUR('',#50776);
#50778=FILL_AREA_STYLE('',(#50777));
#50779=SURFACE_STYLE_FILL_AREA(#50778);
#50780=SURFACE_SIDE_STYLE('',(#50779));
#50781=SURFACE_STYLE_USAGE(.BOTH.,#50780);
#50782=PRESENTATION_STYLE_ASSIGNMENT((#50781));
ENDSEC;
END-ISO-10303-21;
